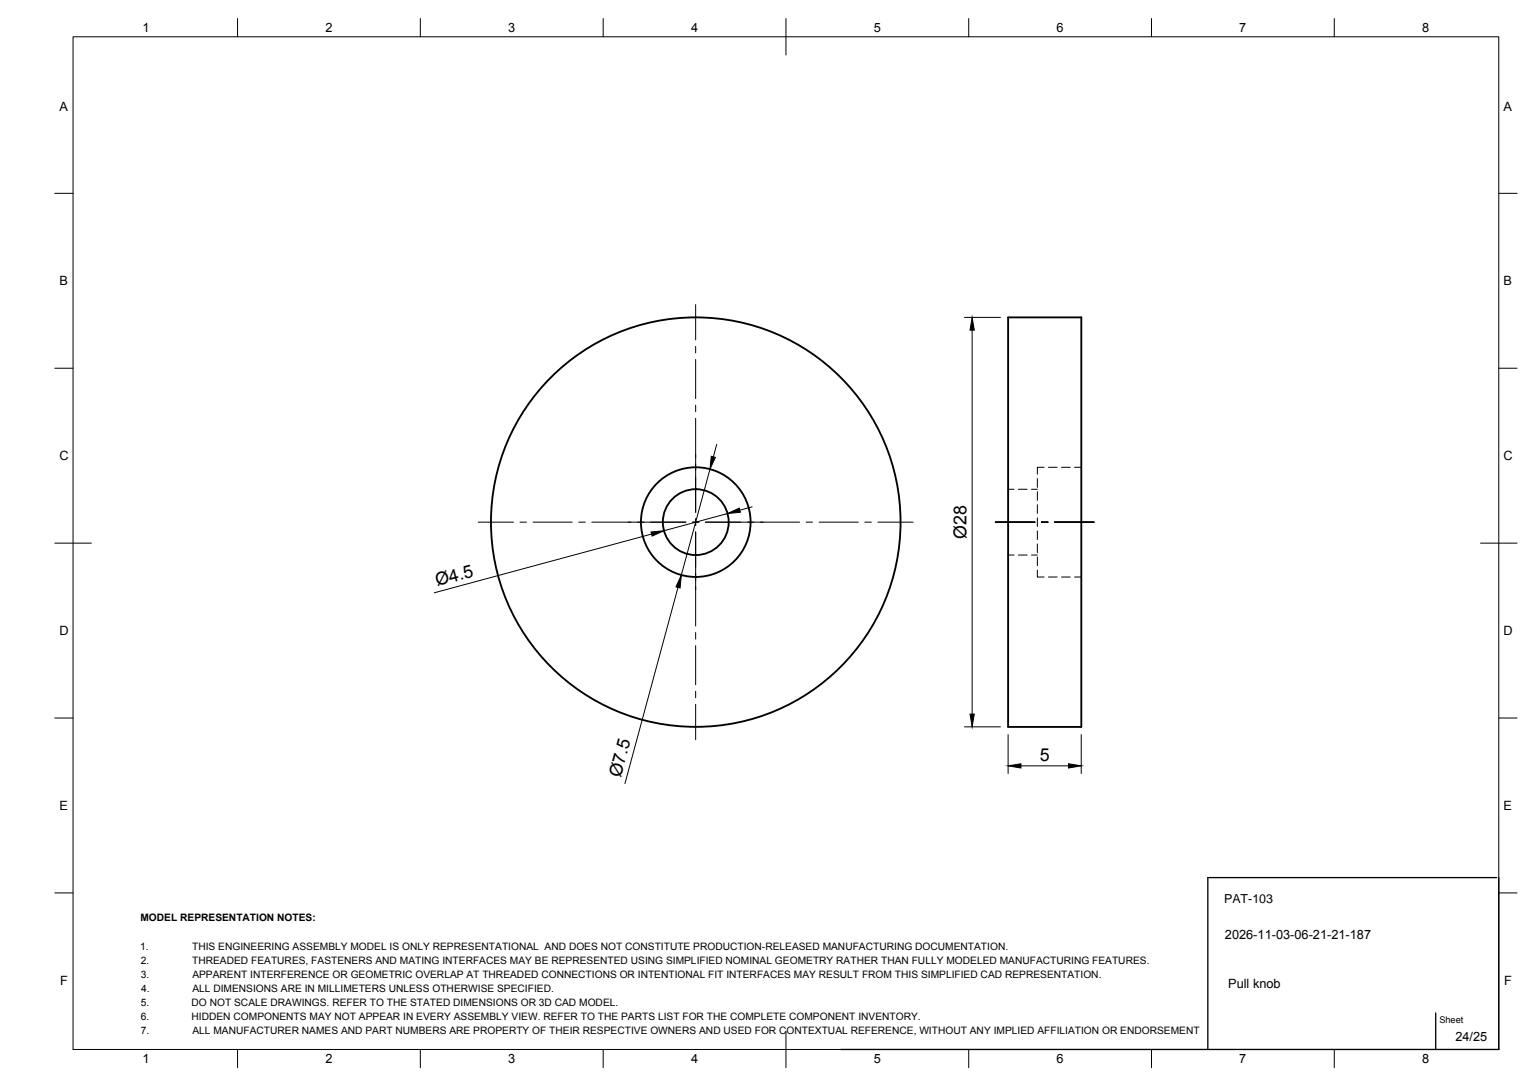
ISO-10303-21;
HEADER;
/* Generated by software containing ST-Developer
 * from STEP Tools, Inc. (www.steptools.com) 
 */

FILE_DESCRIPTION(
/* description */ ('Telescoping shaft support with lock collar'),
/* implementation_level */ '2;1');

FILE_NAME(
/* name */ 'Pull knob.step',
/* time_stamp */ '2026-10-27T10:48:51-07:00',
/* author */ (''),
/* organization */ (''),
/* preprocessor_version */ 'ST-DEVELOPER v20.2',
/* originating_system */ 'Autodesk Translation Framework v15.17.0.0',
/* authorisation */ '');

FILE_SCHEMA (('AUTOMOTIVE_DESIGN { 1 0 10303 214 3 1 1 }'));
ENDSEC;

DATA;
#10=MECHANICAL_DESIGN_GEOMETRIC_PRESENTATION_REPRESENTATION('',(#257),#7349);
#217=SHAPE_REPRESENTATION_RELATIONSHIP('SRR','None',#7461,#237);
#237=ADVANCED_BREP_SHAPE_REPRESENTATION('',(#276),#7345);
#257=STYLED_ITEM('',(#7620),#276);
#276=MANIFOLD_SOLID_BREP('Body1',#3981);
#353=FACE_BOUND('',#981,.T.);
#354=FACE_BOUND('',#985,.T.);
#355=FACE_BOUND('',#987,.T.);
#469=PLANE('',#4604);
#470=PLANE('',#4611);
#471=PLANE('',#4612);
#679=FACE_OUTER_BOUND('',#979,.T.);
#680=FACE_OUTER_BOUND('',#980,.T.);
#681=FACE_OUTER_BOUND('',#982,.T.);
#682=FACE_OUTER_BOUND('',#983,.T.);
#683=FACE_OUTER_BOUND('',#984,.T.);
#684=FACE_OUTER_BOUND('',#986,.T.);
#979=EDGE_LOOP('',(#3508,#3509,#3510,#3511));
#980=EDGE_LOOP('',(#3512));
#981=EDGE_LOOP('',(#3513));
#982=EDGE_LOOP('',(#3514,#3515,#3516,#3517));
#983=EDGE_LOOP('',(#3518,#3519,#3520,#3521));
#984=EDGE_LOOP('',(#3522));
#985=EDGE_LOOP('',(#3523));
#986=EDGE_LOOP('',(#3524));
#987=EDGE_LOOP('',(#3525));
#1255=LINE('',#7098,#1535);
#1256=LINE('',#7105,#1536);
#1257=LINE('',#7111,#1537);
#1535=VECTOR('',#5727,0.375);
#1536=VECTOR('',#5736,0.225);
#1537=VECTOR('',#5743,1.4);
#1774=CIRCLE('',#4602,0.375);
#1775=CIRCLE('',#4603,0.375);
#1776=CIRCLE('',#4605,0.225);
#1777=CIRCLE('',#4607,0.225);
#1778=CIRCLE('',#4609,1.4);
#1779=CIRCLE('',#4610,1.4);
#2085=VERTEX_POINT('',#7095);
#2086=VERTEX_POINT('',#7097);
#2087=VERTEX_POINT('',#7101);
#2088=VERTEX_POINT('',#7104);
#2089=VERTEX_POINT('',#7108);
#2090=VERTEX_POINT('',#7110);
#2566=EDGE_CURVE('',#2085,#2085,#1774,.T.);
#2567=EDGE_CURVE('',#2085,#2086,#1255,.T.);
#2568=EDGE_CURVE('',#2086,#2086,#1775,.T.);
#2569=EDGE_CURVE('',#2087,#2087,#1776,.T.);
#2570=EDGE_CURVE('',#2087,#2088,#1256,.T.);
#2571=EDGE_CURVE('',#2088,#2088,#1777,.T.);
#2572=EDGE_CURVE('',#2089,#2089,#1778,.T.);
#2573=EDGE_CURVE('',#2089,#2090,#1257,.T.);
#2574=EDGE_CURVE('',#2090,#2090,#1779,.T.);
#3508=ORIENTED_EDGE('',*,*,#2566,.F.);
#3509=ORIENTED_EDGE('',*,*,#2567,.T.);
#3510=ORIENTED_EDGE('',*,*,#2568,.F.);
#3511=ORIENTED_EDGE('',*,*,#2567,.F.);
#3512=ORIENTED_EDGE('',*,*,#2566,.T.);
#3513=ORIENTED_EDGE('',*,*,#2569,.F.);
#3514=ORIENTED_EDGE('',*,*,#2569,.T.);
#3515=ORIENTED_EDGE('',*,*,#2570,.T.);
#3516=ORIENTED_EDGE('',*,*,#2571,.T.);
#3517=ORIENTED_EDGE('',*,*,#2570,.F.);
#3518=ORIENTED_EDGE('',*,*,#2572,.F.);
#3519=ORIENTED_EDGE('',*,*,#2573,.T.);
#3520=ORIENTED_EDGE('',*,*,#2574,.T.);
#3521=ORIENTED_EDGE('',*,*,#2573,.F.);
#3522=ORIENTED_EDGE('',*,*,#2572,.T.);
#3523=ORIENTED_EDGE('',*,*,#2568,.T.);
#3524=ORIENTED_EDGE('',*,*,#2574,.F.);
#3525=ORIENTED_EDGE('',*,*,#2571,.F.);
#3730=CYLINDRICAL_SURFACE('',#4601,0.375);
#3731=CYLINDRICAL_SURFACE('',#4606,0.225);
#3732=CYLINDRICAL_SURFACE('',#4608,1.4);
#3922=ADVANCED_FACE('',(#679),#3730,.F.);
#3923=ADVANCED_FACE('',(#680,#353),#469,.T.);
#3924=ADVANCED_FACE('',(#681),#3731,.F.);
#3925=ADVANCED_FACE('',(#682),#3732,.T.);
#3926=ADVANCED_FACE('',(#683,#354),#470,.T.);
#3927=ADVANCED_FACE('',(#684,#355),#471,.F.);
#3981=CLOSED_SHELL('',(#3922,#3923,#3924,#3925,#3926,#3927));
#4600=AXIS2_PLACEMENT_3D('',#7093,#5721,#5722);
#4601=AXIS2_PLACEMENT_3D('',#7094,#5723,#5724);
#4602=AXIS2_PLACEMENT_3D('',#7096,#5725,#5726);
#4603=AXIS2_PLACEMENT_3D('',#7099,#5728,#5729);
#4604=AXIS2_PLACEMENT_3D('',#7100,#5730,#5731);
#4605=AXIS2_PLACEMENT_3D('',#7102,#5732,#5733);
#4606=AXIS2_PLACEMENT_3D('',#7103,#5734,#5735);
#4607=AXIS2_PLACEMENT_3D('',#7106,#5737,#5738);
#4608=AXIS2_PLACEMENT_3D('',#7107,#5739,#5740);
#4609=AXIS2_PLACEMENT_3D('',#7109,#5741,#5742);
#4610=AXIS2_PLACEMENT_3D('',#7112,#5744,#5745);
#4611=AXIS2_PLACEMENT_3D('',#7113,#5746,#5747);
#4612=AXIS2_PLACEMENT_3D('',#7114,#5748,#5749);
#5721=DIRECTION('axis',(0.,0.,1.));
#5722=DIRECTION('refdir',(1.,0.,0.));
#5723=DIRECTION('center_axis',(1.,0.,0.));
#5724=DIRECTION('ref_axis',(0.,0.,-1.));
#5725=DIRECTION('center_axis',(1.,0.,0.));
#5726=DIRECTION('ref_axis',(0.,0.,-1.));
#5727=DIRECTION('',(1.,0.,0.));
#5728=DIRECTION('center_axis',(-1.,0.,0.));
#5729=DIRECTION('ref_axis',(0.,0.,-1.));
#5730=DIRECTION('center_axis',(1.,0.,0.));
#5731=DIRECTION('ref_axis',(0.,0.,-1.));
#5732=DIRECTION('center_axis',(1.,0.,0.));
#5733=DIRECTION('ref_axis',(0.,0.,-1.));
#5734=DIRECTION('center_axis',(1.,0.,0.));
#5735=DIRECTION('ref_axis',(0.,0.,-1.));
#5736=DIRECTION('',(-1.,0.,0.));
#5737=DIRECTION('center_axis',(-1.,0.,0.));
#5738=DIRECTION('ref_axis',(0.,0.,-1.));
#5739=DIRECTION('center_axis',(1.,0.,0.));
#5740=DIRECTION('ref_axis',(0.,0.,-1.));
#5741=DIRECTION('center_axis',(1.,0.,0.));
#5742=DIRECTION('ref_axis',(0.,0.,-1.));
#5743=DIRECTION('',(-1.,0.,0.));
#5744=DIRECTION('center_axis',(1.,0.,0.));
#5745=DIRECTION('ref_axis',(0.,0.,-1.));
#5746=DIRECTION('center_axis',(1.,0.,0.));
#5747=DIRECTION('ref_axis',(0.,0.,-1.));
#5748=DIRECTION('center_axis',(1.,0.,0.));
#5749=DIRECTION('ref_axis',(0.,0.,-1.));
#7093=CARTESIAN_POINT('',(0.,0.,0.));
#7094=CARTESIAN_POINT('Origin',(12.5,0.,3.5));
#7095=CARTESIAN_POINT('',(12.5,-4.59242549680257E-17,3.875));
#7096=CARTESIAN_POINT('Origin',(12.5,0.,3.5));
#7097=CARTESIAN_POINT('',(12.8,4.59242549680257E-17,3.875));
#7098=CARTESIAN_POINT('',(12.5,-4.59242549680257E-17,3.875));
#7099=CARTESIAN_POINT('Origin',(12.8,0.,3.5));
#7100=CARTESIAN_POINT('Origin',(12.5,0.,3.5));
#7101=CARTESIAN_POINT('',(12.5,-2.75545529808155E-17,3.725));
#7102=CARTESIAN_POINT('Origin',(12.5,0.,3.5));
#7103=CARTESIAN_POINT('Origin',(12.3,0.,3.5));
#7104=CARTESIAN_POINT('',(12.3,-2.75545529808155E-17,3.725));
#7105=CARTESIAN_POINT('',(12.3,-2.75545529808155E-17,3.725));
#7106=CARTESIAN_POINT('Origin',(12.3,0.,3.5));
#7107=CARTESIAN_POINT('Origin',(12.3,0.,3.5));
#7108=CARTESIAN_POINT('',(12.8,-1.71450551880629E-16,4.9));
#7109=CARTESIAN_POINT('Origin',(12.8,0.,3.5));
#7110=CARTESIAN_POINT('',(12.3,-1.71450551880629E-16,4.9));
#7111=CARTESIAN_POINT('',(12.3,-1.71450551880629E-16,4.9));
#7112=CARTESIAN_POINT('Origin',(12.3,0.,3.5));
#7113=CARTESIAN_POINT('Origin',(12.8,0.,3.5));
#7114=CARTESIAN_POINT('Origin',(12.3,0.,3.5));
#7320=UNCERTAINTY_MEASURE_WITH_UNIT(LENGTH_MEASURE(0.001),#7350,
'DISTANCE_ACCURACY_VALUE',
'Maximum model space distance between geometric entities at asserted c
onnectivities');
#7324=UNCERTAINTY_MEASURE_WITH_UNIT(LENGTH_MEASURE(0.001),#7350,
'DISTANCE_ACCURACY_VALUE',
'Maximum model space distance between geometric entities at asserted c
onnectivities');
#7345=(
GEOMETRIC_REPRESENTATION_CONTEXT(3)
GLOBAL_UNCERTAINTY_ASSIGNED_CONTEXT((#7320))
GLOBAL_UNIT_ASSIGNED_CONTEXT((#7350,#7352,#7353))
REPRESENTATION_CONTEXT('','3D')
);
#7349=(
GEOMETRIC_REPRESENTATION_CONTEXT(3)
GLOBAL_UNCERTAINTY_ASSIGNED_CONTEXT((#7324))
GLOBAL_UNIT_ASSIGNED_CONTEXT((#7350,#7352,#7353))
REPRESENTATION_CONTEXT('','3D')
);
#7350=(
LENGTH_UNIT()
NAMED_UNIT(*)
SI_UNIT(.CENTI.,.METRE.)
);
#7352=(
NAMED_UNIT(*)
PLANE_ANGLE_UNIT()
SI_UNIT($,.RADIAN.)
);
#7353=(
NAMED_UNIT(*)
SI_UNIT($,.STERADIAN.)
SOLID_ANGLE_UNIT()
);
#7374=SHAPE_DEFINITION_REPRESENTATION(#7400,#7461);
#7400=PRODUCT_DEFINITION_SHAPE('',$,#7486);
#7461=SHAPE_REPRESENTATION('',(#4600),#7345);
#7465=PRODUCT_DEFINITION_CONTEXT('part definition',#7539,'design');
#7486=PRODUCT_DEFINITION('Pull knob','Pull knob',#7510,#7465);
#7510=PRODUCT_DEFINITION_FORMATION('',$,#7561);
#7539=APPLICATION_CONTEXT(
'Core Data for Automotive Mechanical Design Process');
#7540=PRODUCT_CONTEXT('part definition',#7539,'mechanical');
#7561=PRODUCT('Pull knob','Pull knob','Pull knob',(#7540));
#7614=COLOUR_RGB('Sky Blue',0.24,0.69,0.87);
#7615=FILL_AREA_STYLE_COLOUR('',#7614);
#7616=FILL_AREA_STYLE('',(#7615));
#7617=SURFACE_STYLE_FILL_AREA(#7616);
#7618=SURFACE_SIDE_STYLE('',(#7617));
#7619=SURFACE_STYLE_USAGE(.BOTH.,#7618);
#7620=PRESENTATION_STYLE_ASSIGNMENT((#7619));
ENDSEC;
END-ISO-10303-21;
